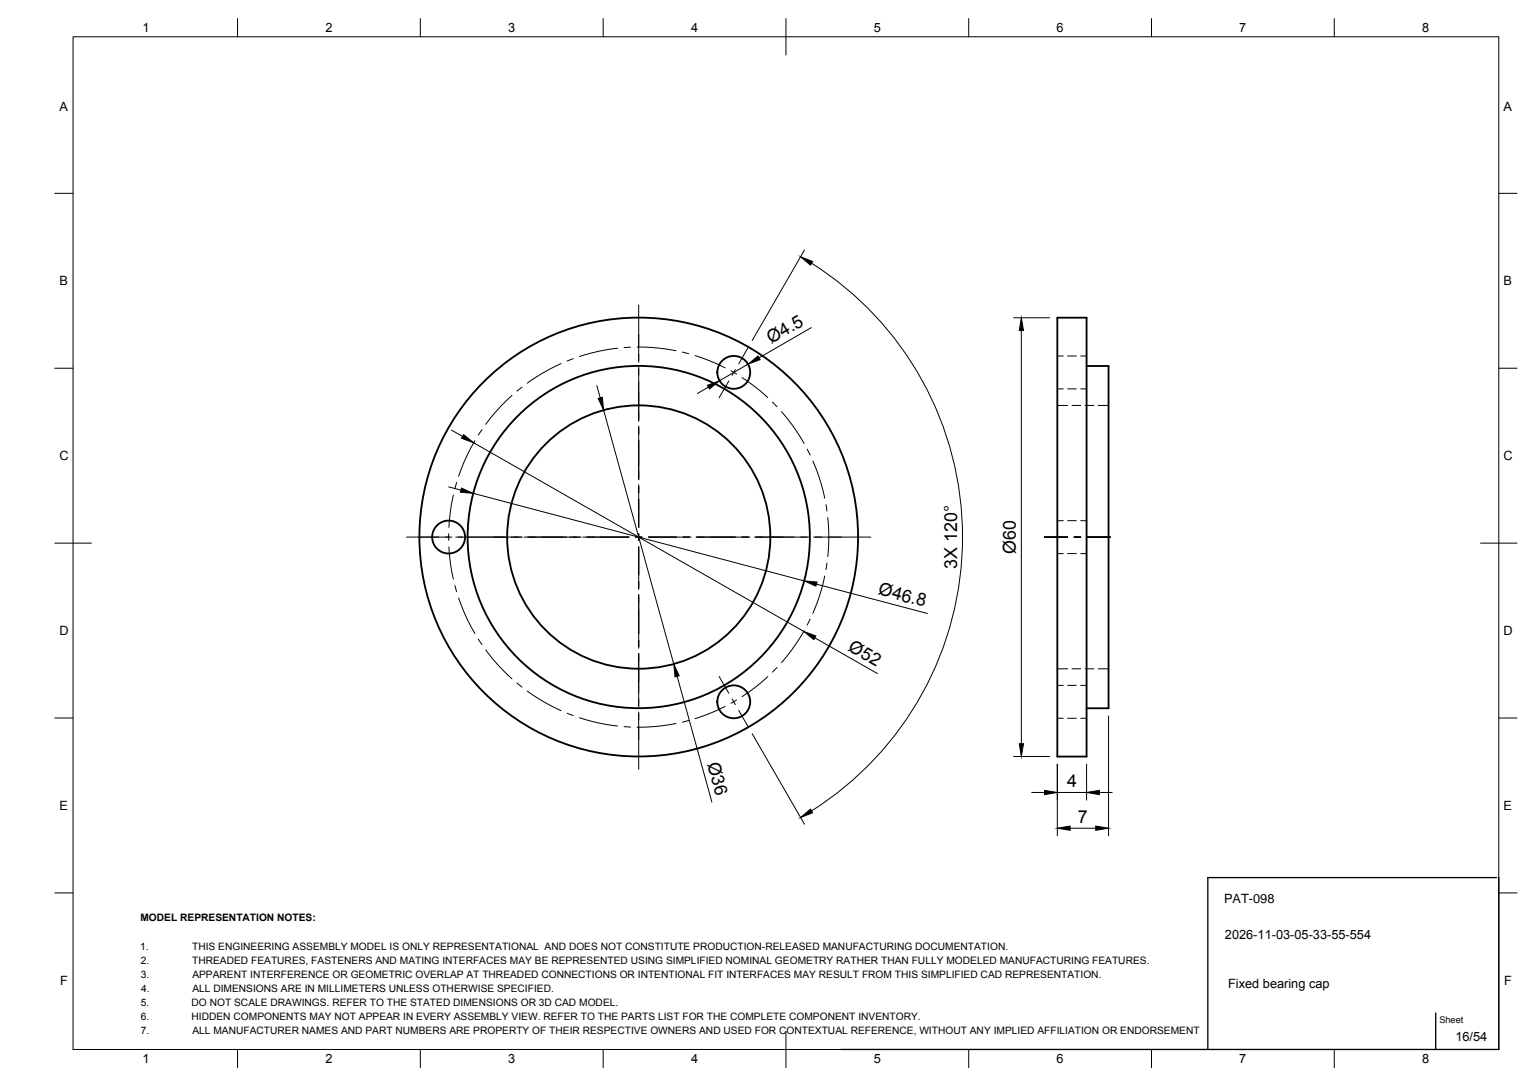
ISO-10303-21;
HEADER;
/* Generated by software containing ST-Developer
 * from STEP Tools, Inc. (www.steptools.com) 
 */

FILE_DESCRIPTION(
/* description */ ('Spring compression tester'),
/* implementation_level */ '2;1');

FILE_NAME(
/* name */ 'Fixed bearing cap.step',
/* time_stamp */ '2026-10-28T03:24:11-07:00',
/* author */ (''),
/* organization */ (''),
/* preprocessor_version */ 'ST-DEVELOPER v20.2',
/* originating_system */ 'Autodesk Translation Framework v15.17.0.0',
/* authorisation */ '');

FILE_SCHEMA (('AUTOMOTIVE_DESIGN { 1 0 10303 214 3 1 1 }'));
ENDSEC;

DATA;
#10=MECHANICAL_DESIGN_GEOMETRIC_PRESENTATION_REPRESENTATION('',(#1117),#43521);
#997=SHAPE_REPRESENTATION_RELATIONSHIP('SRR','None',#43809,#1057);
#1057=ADVANCED_BREP_SHAPE_REPRESENTATION('',(#1192),#43469);
#1117=STYLED_ITEM('',(#44202),#1192);
#1192=MANIFOLD_SOLID_BREP('Body1',#18554);
#1385=FACE_BOUND('',#3565,.T.);
#1386=FACE_BOUND('',#3569,.T.);
#1387=FACE_BOUND('',#3570,.T.);
#1388=FACE_BOUND('',#3571,.T.);
#1389=FACE_BOUND('',#3572,.T.);
#1390=FACE_BOUND('',#3574,.T.);
#1391=FACE_BOUND('',#3575,.T.);
#1392=FACE_BOUND('',#3576,.T.);
#1393=FACE_BOUND('',#3577,.T.);
#1707=PLANE('',#19699);
#1708=PLANE('',#19706);
#1709=PLANE('',#19707);
#2375=FACE_OUTER_BOUND('',#3560,.T.);
#2376=FACE_OUTER_BOUND('',#3561,.T.);
#2377=FACE_OUTER_BOUND('',#3562,.T.);
#2378=FACE_OUTER_BOUND('',#3563,.T.);
#2379=FACE_OUTER_BOUND('',#3564,.T.);
#2380=FACE_OUTER_BOUND('',#3566,.T.);
#2381=FACE_OUTER_BOUND('',#3567,.T.);
#2382=FACE_OUTER_BOUND('',#3568,.T.);
#2383=FACE_OUTER_BOUND('',#3573,.T.);
#3560=EDGE_LOOP('',(#13147,#13148,#13149,#13150));
#3561=EDGE_LOOP('',(#13151,#13152,#13153,#13154));
#3562=EDGE_LOOP('',(#13155,#13156,#13157,#13158));
#3563=EDGE_LOOP('',(#13159,#13160,#13161,#13162));
#3564=EDGE_LOOP('',(#13163));
#3565=EDGE_LOOP('',(#13164));
#3566=EDGE_LOOP('',(#13165,#13166,#13167,#13168));
#3567=EDGE_LOOP('',(#13169,#13170,#13171,#13172));
#3568=EDGE_LOOP('',(#13173));
#3569=EDGE_LOOP('',(#13174));
#3570=EDGE_LOOP('',(#13175));
#3571=EDGE_LOOP('',(#13176));
#3572=EDGE_LOOP('',(#13177));
#3573=EDGE_LOOP('',(#13178));
#3574=EDGE_LOOP('',(#13179));
#3575=EDGE_LOOP('',(#13180));
#3576=EDGE_LOOP('',(#13181));
#3577=EDGE_LOOP('',(#13182));
#4889=LINE('',#27452,#6321);
#4890=LINE('',#27458,#6322);
#4891=LINE('',#27464,#6323);
#4892=LINE('',#27470,#6324);
#4893=LINE('',#27478,#6325);
#4894=LINE('',#27483,#6326);
#6321=VECTOR('',#22289,0.225);
#6322=VECTOR('',#22296,0.225);
#6323=VECTOR('',#22303,0.225);
#6324=VECTOR('',#22310,2.34);
#6325=VECTOR('',#22321,1.8);
#6326=VECTOR('',#22326,3.);
#7652=CIRCLE('',#19688,0.225);
#7653=CIRCLE('',#19689,0.225);
#7654=CIRCLE('',#19691,0.225);
#7655=CIRCLE('',#19692,0.225);
#7656=CIRCLE('',#19694,0.225);
#7657=CIRCLE('',#19695,0.225);
#7658=CIRCLE('',#19697,2.34);
#7659=CIRCLE('',#19698,2.34);
#7660=CIRCLE('',#19700,1.8);
#7661=CIRCLE('',#19702,1.8);
#7662=CIRCLE('',#19704,3.);
#7663=CIRCLE('',#19705,3.);
#8446=VERTEX_POINT('',#27449);
#8447=VERTEX_POINT('',#27451);
#8448=VERTEX_POINT('',#27455);
#8449=VERTEX_POINT('',#27457);
#8450=VERTEX_POINT('',#27461);
#8451=VERTEX_POINT('',#27463);
#8452=VERTEX_POINT('',#27467);
#8453=VERTEX_POINT('',#27469);
#8454=VERTEX_POINT('',#27473);
#8455=VERTEX_POINT('',#27476);
#8456=VERTEX_POINT('',#27480);
#8457=VERTEX_POINT('',#27482);
#10238=EDGE_CURVE('',#8446,#8446,#7652,.T.);
#10239=EDGE_CURVE('',#8446,#8447,#4889,.T.);
#10240=EDGE_CURVE('',#8447,#8447,#7653,.T.);
#10241=EDGE_CURVE('',#8448,#8448,#7654,.T.);
#10242=EDGE_CURVE('',#8448,#8449,#4890,.T.);
#10243=EDGE_CURVE('',#8449,#8449,#7655,.T.);
#10244=EDGE_CURVE('',#8450,#8450,#7656,.T.);
#10245=EDGE_CURVE('',#8450,#8451,#4891,.T.);
#10246=EDGE_CURVE('',#8451,#8451,#7657,.T.);
#10247=EDGE_CURVE('',#8452,#8452,#7658,.T.);
#10248=EDGE_CURVE('',#8452,#8453,#4892,.T.);
#10249=EDGE_CURVE('',#8453,#8453,#7659,.T.);
#10250=EDGE_CURVE('',#8454,#8454,#7660,.T.);
#10251=EDGE_CURVE('',#8455,#8455,#7661,.T.);
#10252=EDGE_CURVE('',#8455,#8454,#4893,.T.);
#10253=EDGE_CURVE('',#8456,#8456,#7662,.T.);
#10254=EDGE_CURVE('',#8456,#8457,#4894,.T.);
#10255=EDGE_CURVE('',#8457,#8457,#7663,.T.);
#13147=ORIENTED_EDGE('',*,*,#10238,.F.);
#13148=ORIENTED_EDGE('',*,*,#10239,.T.);
#13149=ORIENTED_EDGE('',*,*,#10240,.F.);
#13150=ORIENTED_EDGE('',*,*,#10239,.F.);
#13151=ORIENTED_EDGE('',*,*,#10241,.F.);
#13152=ORIENTED_EDGE('',*,*,#10242,.T.);
#13153=ORIENTED_EDGE('',*,*,#10243,.F.);
#13154=ORIENTED_EDGE('',*,*,#10242,.F.);
#13155=ORIENTED_EDGE('',*,*,#10244,.F.);
#13156=ORIENTED_EDGE('',*,*,#10245,.T.);
#13157=ORIENTED_EDGE('',*,*,#10246,.F.);
#13158=ORIENTED_EDGE('',*,*,#10245,.F.);
#13159=ORIENTED_EDGE('',*,*,#10247,.F.);
#13160=ORIENTED_EDGE('',*,*,#10248,.T.);
#13161=ORIENTED_EDGE('',*,*,#10249,.T.);
#13162=ORIENTED_EDGE('',*,*,#10248,.F.);
#13163=ORIENTED_EDGE('',*,*,#10249,.F.);
#13164=ORIENTED_EDGE('',*,*,#10250,.F.);
#13165=ORIENTED_EDGE('',*,*,#10251,.F.);
#13166=ORIENTED_EDGE('',*,*,#10252,.T.);
#13167=ORIENTED_EDGE('',*,*,#10250,.T.);
#13168=ORIENTED_EDGE('',*,*,#10252,.F.);
#13169=ORIENTED_EDGE('',*,*,#10253,.F.);
#13170=ORIENTED_EDGE('',*,*,#10254,.T.);
#13171=ORIENTED_EDGE('',*,*,#10255,.T.);
#13172=ORIENTED_EDGE('',*,*,#10254,.F.);
#13173=ORIENTED_EDGE('',*,*,#10253,.T.);
#13174=ORIENTED_EDGE('',*,*,#10240,.T.);
#13175=ORIENTED_EDGE('',*,*,#10243,.T.);
#13176=ORIENTED_EDGE('',*,*,#10246,.T.);
#13177=ORIENTED_EDGE('',*,*,#10251,.T.);
#13178=ORIENTED_EDGE('',*,*,#10255,.F.);
#13179=ORIENTED_EDGE('',*,*,#10238,.T.);
#13180=ORIENTED_EDGE('',*,*,#10241,.T.);
#13181=ORIENTED_EDGE('',*,*,#10244,.T.);
#13182=ORIENTED_EDGE('',*,*,#10247,.T.);
#17192=CYLINDRICAL_SURFACE('',#19687,0.225);
#17193=CYLINDRICAL_SURFACE('',#19690,0.225);
#17194=CYLINDRICAL_SURFACE('',#19693,0.225);
#17195=CYLINDRICAL_SURFACE('',#19696,2.34);
#17196=CYLINDRICAL_SURFACE('',#19701,1.8);
#17197=CYLINDRICAL_SURFACE('',#19703,3.);
#17699=ADVANCED_FACE('',(#2375),#17192,.F.);
#17700=ADVANCED_FACE('',(#2376),#17193,.F.);
#17701=ADVANCED_FACE('',(#2377),#17194,.F.);
#17702=ADVANCED_FACE('',(#2378),#17195,.T.);
#17703=ADVANCED_FACE('',(#2379,#1385),#1707,.F.);
#17704=ADVANCED_FACE('',(#2380),#17196,.F.);
#17705=ADVANCED_FACE('',(#2381),#17197,.T.);
#17706=ADVANCED_FACE('',(#2382,#1386,#1387,#1388,#1389),#1708,.T.);
#17707=ADVANCED_FACE('',(#2383,#1390,#1391,#1392,#1393),#1709,.F.);
#18554=CLOSED_SHELL('',(#17699,#17700,#17701,#17702,#17703,#17704,#17705,
#17706,#17707));
#19686=AXIS2_PLACEMENT_3D('',#27447,#22283,#22284);
#19687=AXIS2_PLACEMENT_3D('',#27448,#22285,#22286);
#19688=AXIS2_PLACEMENT_3D('',#27450,#22287,#22288);
#19689=AXIS2_PLACEMENT_3D('',#27453,#22290,#22291);
#19690=AXIS2_PLACEMENT_3D('',#27454,#22292,#22293);
#19691=AXIS2_PLACEMENT_3D('',#27456,#22294,#22295);
#19692=AXIS2_PLACEMENT_3D('',#27459,#22297,#22298);
#19693=AXIS2_PLACEMENT_3D('',#27460,#22299,#22300);
#19694=AXIS2_PLACEMENT_3D('',#27462,#22301,#22302);
#19695=AXIS2_PLACEMENT_3D('',#27465,#22304,#22305);
#19696=AXIS2_PLACEMENT_3D('',#27466,#22306,#22307);
#19697=AXIS2_PLACEMENT_3D('',#27468,#22308,#22309);
#19698=AXIS2_PLACEMENT_3D('',#27471,#22311,#22312);
#19699=AXIS2_PLACEMENT_3D('',#27472,#22313,#22314);
#19700=AXIS2_PLACEMENT_3D('',#27474,#22315,#22316);
#19701=AXIS2_PLACEMENT_3D('',#27475,#22317,#22318);
#19702=AXIS2_PLACEMENT_3D('',#27477,#22319,#22320);
#19703=AXIS2_PLACEMENT_3D('',#27479,#22322,#22323);
#19704=AXIS2_PLACEMENT_3D('',#27481,#22324,#22325);
#19705=AXIS2_PLACEMENT_3D('',#27484,#22327,#22328);
#19706=AXIS2_PLACEMENT_3D('',#27485,#22329,#22330);
#19707=AXIS2_PLACEMENT_3D('',#27486,#22331,#22332);
#22283=DIRECTION('axis',(0.,0.,1.));
#22284=DIRECTION('refdir',(1.,0.,0.));
#22285=DIRECTION('center_axis',(0.,0.,1.));
#22286=DIRECTION('ref_axis',(1.,0.,0.));
#22287=DIRECTION('center_axis',(0.,0.,1.));
#22288=DIRECTION('ref_axis',(1.,0.,0.));
#22289=DIRECTION('',(0.,0.,1.));
#22290=DIRECTION('center_axis',(0.,0.,-1.));
#22291=DIRECTION('ref_axis',(1.,0.,0.));
#22292=DIRECTION('center_axis',(0.,0.,1.));
#22293=DIRECTION('ref_axis',(1.,0.,0.));
#22294=DIRECTION('center_axis',(0.,0.,1.));
#22295=DIRECTION('ref_axis',(1.,0.,0.));
#22296=DIRECTION('',(0.,0.,1.));
#22297=DIRECTION('center_axis',(0.,0.,-1.));
#22298=DIRECTION('ref_axis',(1.,0.,0.));
#22299=DIRECTION('center_axis',(0.,0.,1.));
#22300=DIRECTION('ref_axis',(1.,0.,0.));
#22301=DIRECTION('center_axis',(0.,0.,1.));
#22302=DIRECTION('ref_axis',(1.,0.,0.));
#22303=DIRECTION('',(0.,0.,1.));
#22304=DIRECTION('center_axis',(0.,0.,-1.));
#22305=DIRECTION('ref_axis',(1.,0.,0.));
#22306=DIRECTION('center_axis',(0.,0.,1.));
#22307=DIRECTION('ref_axis',(1.,0.,0.));
#22308=DIRECTION('center_axis',(0.,0.,1.));
#22309=DIRECTION('ref_axis',(1.,0.,0.));
#22310=DIRECTION('',(0.,0.,-1.));
#22311=DIRECTION('center_axis',(0.,0.,1.));
#22312=DIRECTION('ref_axis',(1.,0.,0.));
#22313=DIRECTION('center_axis',(0.,0.,1.));
#22314=DIRECTION('ref_axis',(1.,0.,0.));
#22315=DIRECTION('center_axis',(0.,0.,-1.));
#22316=DIRECTION('ref_axis',(1.,0.,0.));
#22317=DIRECTION('center_axis',(0.,0.,1.));
#22318=DIRECTION('ref_axis',(1.,0.,0.));
#22319=DIRECTION('center_axis',(0.,0.,-1.));
#22320=DIRECTION('ref_axis',(1.,0.,0.));
#22321=DIRECTION('',(0.,0.,-1.));
#22322=DIRECTION('center_axis',(0.,0.,1.));
#22323=DIRECTION('ref_axis',(1.,0.,0.));
#22324=DIRECTION('center_axis',(0.,0.,1.));
#22325=DIRECTION('ref_axis',(1.,0.,0.));
#22326=DIRECTION('',(0.,0.,-1.));
#22327=DIRECTION('center_axis',(0.,0.,1.));
#22328=DIRECTION('ref_axis',(1.,0.,0.));
#22329=DIRECTION('center_axis',(0.,0.,1.));
#22330=DIRECTION('ref_axis',(1.,0.,0.));
#22331=DIRECTION('center_axis',(0.,0.,1.));
#22332=DIRECTION('ref_axis',(1.,0.,0.));
#27447=CARTESIAN_POINT('',(0.,0.,0.));
#27448=CARTESIAN_POINT('Origin',(2.6,5.,24.9));
#27449=CARTESIAN_POINT('',(2.375,5.,25.));
#27450=CARTESIAN_POINT('Origin',(2.6,5.,25.));
#27451=CARTESIAN_POINT('',(2.375,5.,25.4));
#27452=CARTESIAN_POINT('',(2.375,5.,24.9));
#27453=CARTESIAN_POINT('Origin',(2.6,5.,25.4));
#27454=CARTESIAN_POINT('Origin',(-1.3,7.25166604983954,24.9));
#27455=CARTESIAN_POINT('',(-1.525,7.25166604983954,25.));
#27456=CARTESIAN_POINT('Origin',(-1.3,7.25166604983954,25.));
#27457=CARTESIAN_POINT('',(-1.525,7.25166604983954,25.4));
#27458=CARTESIAN_POINT('',(-1.525,7.25166604983954,24.9));
#27459=CARTESIAN_POINT('Origin',(-1.3,7.25166604983954,25.4));
#27460=CARTESIAN_POINT('Origin',(-1.3,2.74833395016046,24.9));
#27461=CARTESIAN_POINT('',(-1.525,2.74833395016046,25.));
#27462=CARTESIAN_POINT('Origin',(-1.3,2.74833395016046,25.));
#27463=CARTESIAN_POINT('',(-1.525,2.74833395016046,25.4));
#27464=CARTESIAN_POINT('',(-1.525,2.74833395016046,24.9));
#27465=CARTESIAN_POINT('Origin',(-1.3,2.74833395016046,25.4));
#27466=CARTESIAN_POINT('Origin',(0.,5.,24.7));
#27467=CARTESIAN_POINT('',(-2.34,5.,25.));
#27468=CARTESIAN_POINT('Origin',(0.,5.,25.));
#27469=CARTESIAN_POINT('',(-2.34,5.,24.7));
#27470=CARTESIAN_POINT('',(-2.34,5.,24.7));
#27471=CARTESIAN_POINT('Origin',(0.,5.,24.7));
#27472=CARTESIAN_POINT('Origin',(0.,5.,24.7));
#27473=CARTESIAN_POINT('',(-1.8,5.,24.7));
#27474=CARTESIAN_POINT('Origin',(0.,5.,24.7));
#27475=CARTESIAN_POINT('Origin',(0.,5.,25.));
#27476=CARTESIAN_POINT('',(-1.8,5.,25.4));
#27477=CARTESIAN_POINT('Origin',(0.,5.,25.4));
#27478=CARTESIAN_POINT('',(-1.8,5.,25.));
#27479=CARTESIAN_POINT('Origin',(0.,5.,25.));
#27480=CARTESIAN_POINT('',(-3.,5.,25.4));
#27481=CARTESIAN_POINT('Origin',(0.,5.,25.4));
#27482=CARTESIAN_POINT('',(-3.,5.,25.));
#27483=CARTESIAN_POINT('',(-3.,5.,25.));
#27484=CARTESIAN_POINT('Origin',(0.,5.,25.));
#27485=CARTESIAN_POINT('Origin',(0.,5.,25.4));
#27486=CARTESIAN_POINT('Origin',(0.,5.,25.));
#43401=UNCERTAINTY_MEASURE_WITH_UNIT(LENGTH_MEASURE(0.001),#43522,
'DISTANCE_ACCURACY_VALUE',
'Maximum model space distance between geometric entities at asserted c
onnectivities');
#43453=UNCERTAINTY_MEASURE_WITH_UNIT(LENGTH_MEASURE(0.001),#43522,
'DISTANCE_ACCURACY_VALUE',
'Maximum model space distance between geometric entities at asserted c
onnectivities');
#43469=(
GEOMETRIC_REPRESENTATION_CONTEXT(3)
GLOBAL_UNCERTAINTY_ASSIGNED_CONTEXT((#43401))
GLOBAL_UNIT_ASSIGNED_CONTEXT((#43522,#43524,#43525))
REPRESENTATION_CONTEXT('','3D')
);
#43521=(
GEOMETRIC_REPRESENTATION_CONTEXT(3)
GLOBAL_UNCERTAINTY_ASSIGNED_CONTEXT((#43453))
GLOBAL_UNIT_ASSIGNED_CONTEXT((#43522,#43524,#43525))
REPRESENTATION_CONTEXT('','3D')
);
#43522=(
LENGTH_UNIT()
NAMED_UNIT(*)
SI_UNIT(.CENTI.,.METRE.)
);
#43524=(
NAMED_UNIT(*)
PLANE_ANGLE_UNIT()
SI_UNIT($,.RADIAN.)
);
#43525=(
NAMED_UNIT(*)
SI_UNIT($,.STERADIAN.)
SOLID_ANGLE_UNIT()
);
#43541=SHAPE_DEFINITION_REPRESENTATION(#43608,#43809);
#43608=PRODUCT_DEFINITION_SHAPE('',$,#43877);
#43809=SHAPE_REPRESENTATION('',(#19686),#43469);
#43861=PRODUCT_DEFINITION_CONTEXT('part definition',#44064,'design');
#43877=PRODUCT_DEFINITION('Fixed bearing cap','Fixed bearing cap',#43944,
#43861);
#43944=PRODUCT_DEFINITION_FORMATION('',$,#44081);
#44064=APPLICATION_CONTEXT(
'Core Data for Automotive Mechanical Design Process');
#44065=PRODUCT_CONTEXT('part definition',#44064,'mechanical');
#44081=PRODUCT('Fixed bearing cap','Fixed bearing cap',
'Fixed bearing cap',(#44065));
#44196=COLOUR_RGB('Grey',0.48,0.52,0.57);
#44197=FILL_AREA_STYLE_COLOUR('',#44196);
#44198=FILL_AREA_STYLE('',(#44197));
#44199=SURFACE_STYLE_FILL_AREA(#44198);
#44200=SURFACE_SIDE_STYLE('',(#44199));
#44201=SURFACE_STYLE_USAGE(.BOTH.,#44200);
#44202=PRESENTATION_STYLE_ASSIGNMENT((#44201));
ENDSEC;
END-ISO-10303-21;
